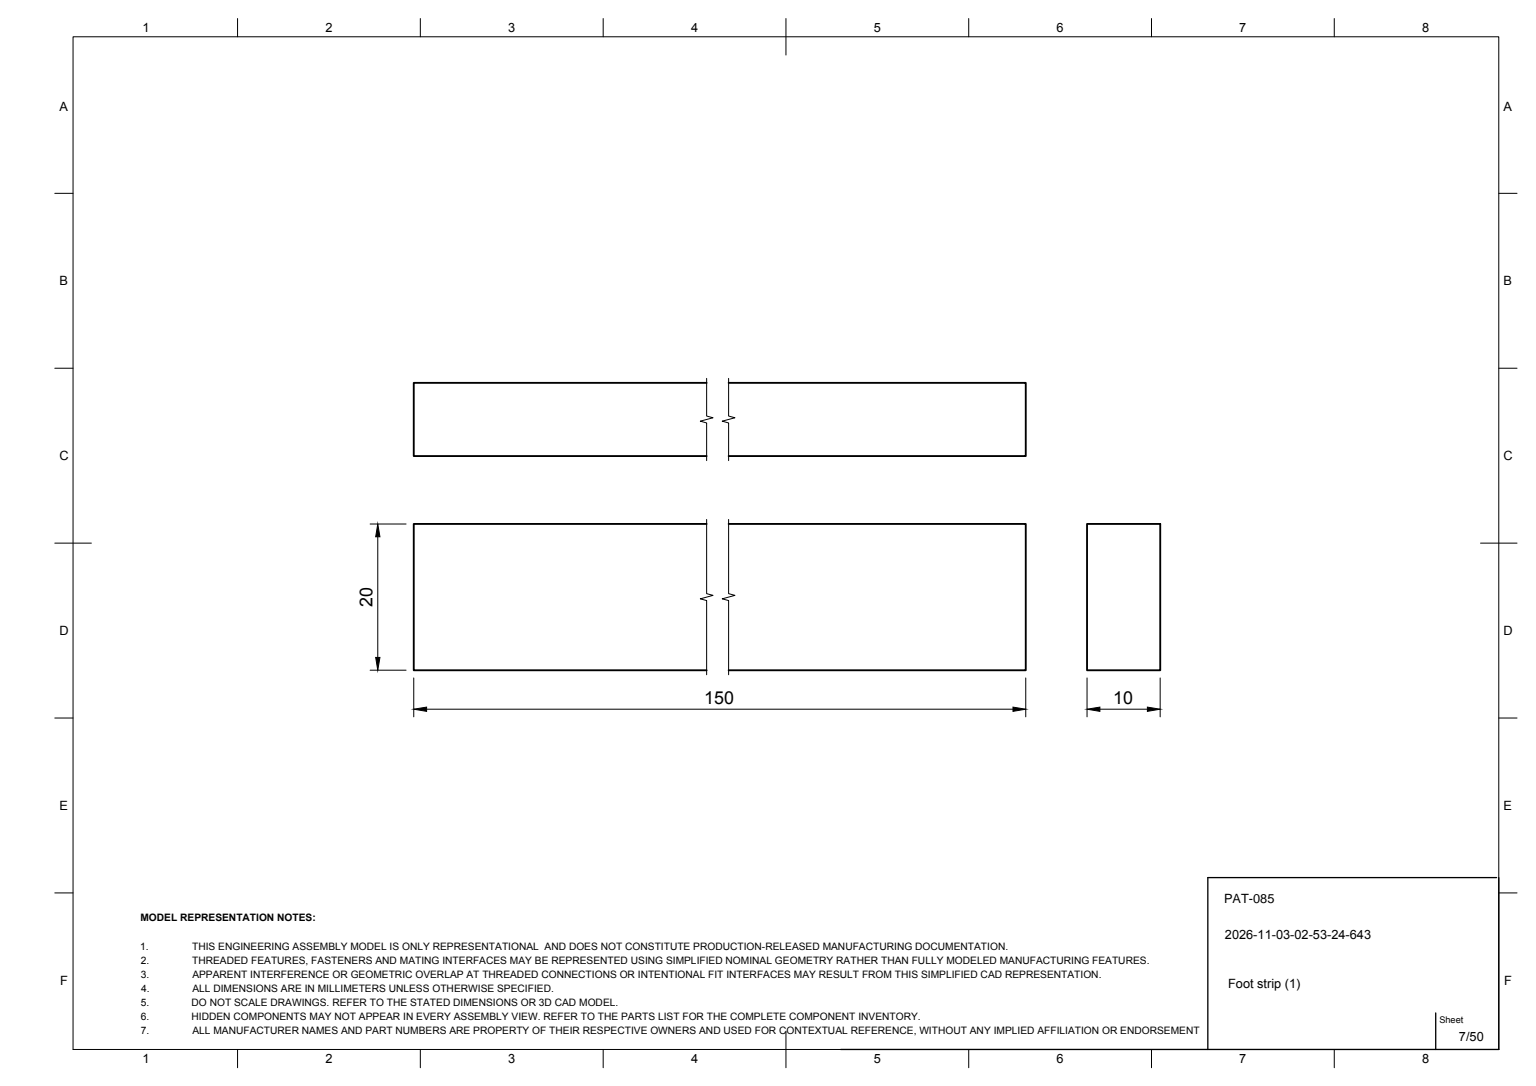
ISO-10303-21;
HEADER;
/* Generated by software containing ST-Developer
 * from STEP Tools, Inc. (www.steptools.com) 
 */

FILE_DESCRIPTION(
/* description */ ('Rack and pinion manual slide'),
/* implementation_level */ '2;1');

FILE_NAME(
/* name */ 'Foot strip (1).step',
/* time_stamp */ '2026-10-28T03:22:49-07:00',
/* author */ (''),
/* organization */ (''),
/* preprocessor_version */ 'ST-DEVELOPER v20.2',
/* originating_system */ 'Autodesk Translation Framework v15.17.0.0',
/* authorisation */ '');

FILE_SCHEMA (('AUTOMOTIVE_DESIGN { 1 0 10303 214 3 1 1 }'));
ENDSEC;

DATA;
#10=MECHANICAL_DESIGN_GEOMETRIC_PRESENTATION_REPRESENTATION('',(#734),#34851);
#642=SHAPE_REPRESENTATION_RELATIONSHIP('SRR','None',#35077,#688);
#688=ADVANCED_BREP_SHAPE_REPRESENTATION('',(#787),#34802);
#734=STYLED_ITEM('',(#35397),#787);
#787=MANIFOLD_SOLID_BREP('Body1',#13754);
#1056=PLANE('',#14346);
#1057=PLANE('',#14347);
#1058=PLANE('',#14348);
#1059=PLANE('',#14349);
#1060=PLANE('',#14350);
#1061=PLANE('',#14351);
#1551=FACE_OUTER_BOUND('',#2298,.T.);
#1552=FACE_OUTER_BOUND('',#2299,.T.);
#1553=FACE_OUTER_BOUND('',#2300,.T.);
#1554=FACE_OUTER_BOUND('',#2301,.T.);
#1555=FACE_OUTER_BOUND('',#2302,.T.);
#1556=FACE_OUTER_BOUND('',#2303,.T.);
#2298=EDGE_LOOP('',(#9306,#9307,#9308,#9309));
#2299=EDGE_LOOP('',(#9310,#9311,#9312,#9313));
#2300=EDGE_LOOP('',(#9314,#9315,#9316,#9317));
#2301=EDGE_LOOP('',(#9318,#9319,#9320,#9321));
#2302=EDGE_LOOP('',(#9322,#9323,#9324,#9325));
#2303=EDGE_LOOP('',(#9326,#9327,#9328,#9329));
#3252=LINE('',#19541,#4543);
#3253=LINE('',#19543,#4544);
#3254=LINE('',#19545,#4545);
#3255=LINE('',#19546,#4546);
#3256=LINE('',#19549,#4547);
#3257=LINE('',#19551,#4548);
#3258=LINE('',#19552,#4549);
#3259=LINE('',#19555,#4550);
#3260=LINE('',#19557,#4551);
#3261=LINE('',#19558,#4552);
#3262=LINE('',#19560,#4553);
#3263=LINE('',#19561,#4554);
#4543=VECTOR('',#15688,1.);
#4544=VECTOR('',#15689,1.);
#4545=VECTOR('',#15690,1.);
#4546=VECTOR('',#15691,1.);
#4547=VECTOR('',#15694,1.);
#4548=VECTOR('',#15695,1.);
#4549=VECTOR('',#15696,1.);
#4550=VECTOR('',#15699,1.);
#4551=VECTOR('',#15700,1.);
#4552=VECTOR('',#15701,1.);
#4553=VECTOR('',#15704,1.);
#4554=VECTOR('',#15705,1.);
#6248=VERTEX_POINT('',#19539);
#6249=VERTEX_POINT('',#19540);
#6250=VERTEX_POINT('',#19542);
#6251=VERTEX_POINT('',#19544);
#6252=VERTEX_POINT('',#19548);
#6253=VERTEX_POINT('',#19550);
#6254=VERTEX_POINT('',#19554);
#6255=VERTEX_POINT('',#19556);
#7465=EDGE_CURVE('',#6248,#6249,#3252,.T.);
#7466=EDGE_CURVE('',#6249,#6250,#3253,.T.);
#7467=EDGE_CURVE('',#6251,#6250,#3254,.T.);
#7468=EDGE_CURVE('',#6248,#6251,#3255,.T.);
#7469=EDGE_CURVE('',#6252,#6248,#3256,.T.);
#7470=EDGE_CURVE('',#6253,#6251,#3257,.T.);
#7471=EDGE_CURVE('',#6252,#6253,#3258,.T.);
#7472=EDGE_CURVE('',#6254,#6252,#3259,.T.);
#7473=EDGE_CURVE('',#6255,#6253,#3260,.T.);
#7474=EDGE_CURVE('',#6254,#6255,#3261,.T.);
#7475=EDGE_CURVE('',#6249,#6254,#3262,.T.);
#7476=EDGE_CURVE('',#6250,#6255,#3263,.T.);
#9306=ORIENTED_EDGE('',*,*,#7465,.T.);
#9307=ORIENTED_EDGE('',*,*,#7466,.T.);
#9308=ORIENTED_EDGE('',*,*,#7467,.F.);
#9309=ORIENTED_EDGE('',*,*,#7468,.F.);
#9310=ORIENTED_EDGE('',*,*,#7469,.T.);
#9311=ORIENTED_EDGE('',*,*,#7468,.T.);
#9312=ORIENTED_EDGE('',*,*,#7470,.F.);
#9313=ORIENTED_EDGE('',*,*,#7471,.F.);
#9314=ORIENTED_EDGE('',*,*,#7472,.T.);
#9315=ORIENTED_EDGE('',*,*,#7471,.T.);
#9316=ORIENTED_EDGE('',*,*,#7473,.F.);
#9317=ORIENTED_EDGE('',*,*,#7474,.F.);
#9318=ORIENTED_EDGE('',*,*,#7475,.T.);
#9319=ORIENTED_EDGE('',*,*,#7474,.T.);
#9320=ORIENTED_EDGE('',*,*,#7476,.F.);
#9321=ORIENTED_EDGE('',*,*,#7466,.F.);
#9322=ORIENTED_EDGE('',*,*,#7476,.T.);
#9323=ORIENTED_EDGE('',*,*,#7473,.T.);
#9324=ORIENTED_EDGE('',*,*,#7470,.T.);
#9325=ORIENTED_EDGE('',*,*,#7467,.T.);
#9326=ORIENTED_EDGE('',*,*,#7475,.F.);
#9327=ORIENTED_EDGE('',*,*,#7465,.F.);
#9328=ORIENTED_EDGE('',*,*,#7469,.F.);
#9329=ORIENTED_EDGE('',*,*,#7472,.F.);
#13029=ADVANCED_FACE('',(#1551),#1056,.T.);
#13030=ADVANCED_FACE('',(#1552),#1057,.T.);
#13031=ADVANCED_FACE('',(#1553),#1058,.T.);
#13032=ADVANCED_FACE('',(#1554),#1059,.T.);
#13033=ADVANCED_FACE('',(#1555),#1060,.T.);
#13034=ADVANCED_FACE('',(#1556),#1061,.F.);
#13754=CLOSED_SHELL('',(#13029,#13030,#13031,#13032,#13033,#13034));
#14345=AXIS2_PLACEMENT_3D('',#19537,#15684,#15685);
#14346=AXIS2_PLACEMENT_3D('',#19538,#15686,#15687);
#14347=AXIS2_PLACEMENT_3D('',#19547,#15692,#15693);
#14348=AXIS2_PLACEMENT_3D('',#19553,#15697,#15698);
#14349=AXIS2_PLACEMENT_3D('',#19559,#15702,#15703);
#14350=AXIS2_PLACEMENT_3D('',#19562,#15706,#15707);
#14351=AXIS2_PLACEMENT_3D('',#19563,#15708,#15709);
#15684=DIRECTION('axis',(0.,0.,1.));
#15685=DIRECTION('refdir',(1.,0.,0.));
#15686=DIRECTION('center_axis',(0.,1.,0.));
#15687=DIRECTION('ref_axis',(-1.,0.,0.));
#15688=DIRECTION('',(-1.,0.,0.));
#15689=DIRECTION('',(0.,0.,1.));
#15690=DIRECTION('',(-1.,0.,0.));
#15691=DIRECTION('',(0.,0.,1.));
#15692=DIRECTION('center_axis',(1.,0.,0.));
#15693=DIRECTION('ref_axis',(0.,1.,0.));
#15694=DIRECTION('',(0.,1.,0.));
#15695=DIRECTION('',(0.,1.,0.));
#15696=DIRECTION('',(0.,0.,1.));
#15697=DIRECTION('center_axis',(0.,-1.,0.));
#15698=DIRECTION('ref_axis',(1.,0.,0.));
#15699=DIRECTION('',(1.,0.,0.));
#15700=DIRECTION('',(1.,0.,0.));
#15701=DIRECTION('',(0.,0.,1.));
#15702=DIRECTION('center_axis',(-1.,0.,0.));
#15703=DIRECTION('ref_axis',(0.,-1.,0.));
#15704=DIRECTION('',(0.,-1.,0.));
#15705=DIRECTION('',(0.,-1.,0.));
#15706=DIRECTION('center_axis',(0.,0.,1.));
#15707=DIRECTION('ref_axis',(1.,0.,0.));
#15708=DIRECTION('center_axis',(0.,0.,1.));
#15709=DIRECTION('ref_axis',(1.,0.,0.));
#19537=CARTESIAN_POINT('',(0.,0.,0.));
#19538=CARTESIAN_POINT('Origin',(28.,7.5,-1.));
#19539=CARTESIAN_POINT('',(28.,7.5,-1.));
#19540=CARTESIAN_POINT('',(26.,7.5,-1.));
#19541=CARTESIAN_POINT('',(28.,7.5,-1.));
#19542=CARTESIAN_POINT('',(26.,7.5,0.));
#19543=CARTESIAN_POINT('',(26.,7.5,-1.));
#19544=CARTESIAN_POINT('',(28.,7.5,0.));
#19545=CARTESIAN_POINT('',(28.,7.5,0.));
#19546=CARTESIAN_POINT('',(28.,7.5,-1.));
#19547=CARTESIAN_POINT('Origin',(28.,-7.5,-1.));
#19548=CARTESIAN_POINT('',(28.,-7.5,-1.));
#19549=CARTESIAN_POINT('',(28.,-7.5,-1.));
#19550=CARTESIAN_POINT('',(28.,-7.5,0.));
#19551=CARTESIAN_POINT('',(28.,-7.5,0.));
#19552=CARTESIAN_POINT('',(28.,-7.5,-1.));
#19553=CARTESIAN_POINT('Origin',(26.,-7.5,-1.));
#19554=CARTESIAN_POINT('',(26.,-7.5,-1.));
#19555=CARTESIAN_POINT('',(26.,-7.5,-1.));
#19556=CARTESIAN_POINT('',(26.,-7.5,0.));
#19557=CARTESIAN_POINT('',(26.,-7.5,0.));
#19558=CARTESIAN_POINT('',(26.,-7.5,-1.));
#19559=CARTESIAN_POINT('Origin',(26.,7.5,-1.));
#19560=CARTESIAN_POINT('',(26.,7.5,-1.));
#19561=CARTESIAN_POINT('',(26.,7.5,0.));
#19562=CARTESIAN_POINT('Origin',(27.,0.,0.));
#19563=CARTESIAN_POINT('Origin',(27.,0.,-1.));
#34748=UNCERTAINTY_MEASURE_WITH_UNIT(LENGTH_MEASURE(0.001),#34852,
'DISTANCE_ACCURACY_VALUE',
'Maximum model space distance between geometric entities at asserted c
onnectivities');
#34797=UNCERTAINTY_MEASURE_WITH_UNIT(LENGTH_MEASURE(0.001),#34852,
'DISTANCE_ACCURACY_VALUE',
'Maximum model space distance between geometric entities at asserted c
onnectivities');
#34802=(
GEOMETRIC_REPRESENTATION_CONTEXT(3)
GLOBAL_UNCERTAINTY_ASSIGNED_CONTEXT((#34748))
GLOBAL_UNIT_ASSIGNED_CONTEXT((#34852,#34854,#34855))
REPRESENTATION_CONTEXT('','3D')
);
#34851=(
GEOMETRIC_REPRESENTATION_CONTEXT(3)
GLOBAL_UNCERTAINTY_ASSIGNED_CONTEXT((#34797))
GLOBAL_UNIT_ASSIGNED_CONTEXT((#34852,#34854,#34855))
REPRESENTATION_CONTEXT('','3D')
);
#34852=(
LENGTH_UNIT()
NAMED_UNIT(*)
SI_UNIT(.CENTI.,.METRE.)
);
#34854=(
NAMED_UNIT(*)
PLANE_ANGLE_UNIT()
SI_UNIT($,.RADIAN.)
);
#34855=(
NAMED_UNIT(*)
SI_UNIT($,.STERADIAN.)
SOLID_ANGLE_UNIT()
);
#34860=SHAPE_DEFINITION_REPRESENTATION(#34913,#35077);
#34913=PRODUCT_DEFINITION_SHAPE('',$,#35131);
#35077=SHAPE_REPRESENTATION('',(#14345),#34802);
#35126=PRODUCT_DEFINITION_CONTEXT('part definition',#35287,'design');
#35131=PRODUCT_DEFINITION('Foot strip (1)','Foot strip (1)',#35184,#35126);
#35184=PRODUCT_DEFINITION_FORMATION('',$,#35293);
#35287=APPLICATION_CONTEXT(
'Core Data for Automotive Mechanical Design Process');
#35288=PRODUCT_CONTEXT('part definition',#35287,'mechanical');
#35293=PRODUCT('Foot strip (1)','Foot strip (1)','Foot strip (1)',(#35288));
#35391=COLOUR_RGB('Light Blue',0.38,0.62,0.78);
#35392=FILL_AREA_STYLE_COLOUR('',#35391);
#35393=FILL_AREA_STYLE('',(#35392));
#35394=SURFACE_STYLE_FILL_AREA(#35393);
#35395=SURFACE_SIDE_STYLE('',(#35394));
#35396=SURFACE_STYLE_USAGE(.BOTH.,#35395);
#35397=PRESENTATION_STYLE_ASSIGNMENT((#35396));
ENDSEC;
END-ISO-10303-21;
